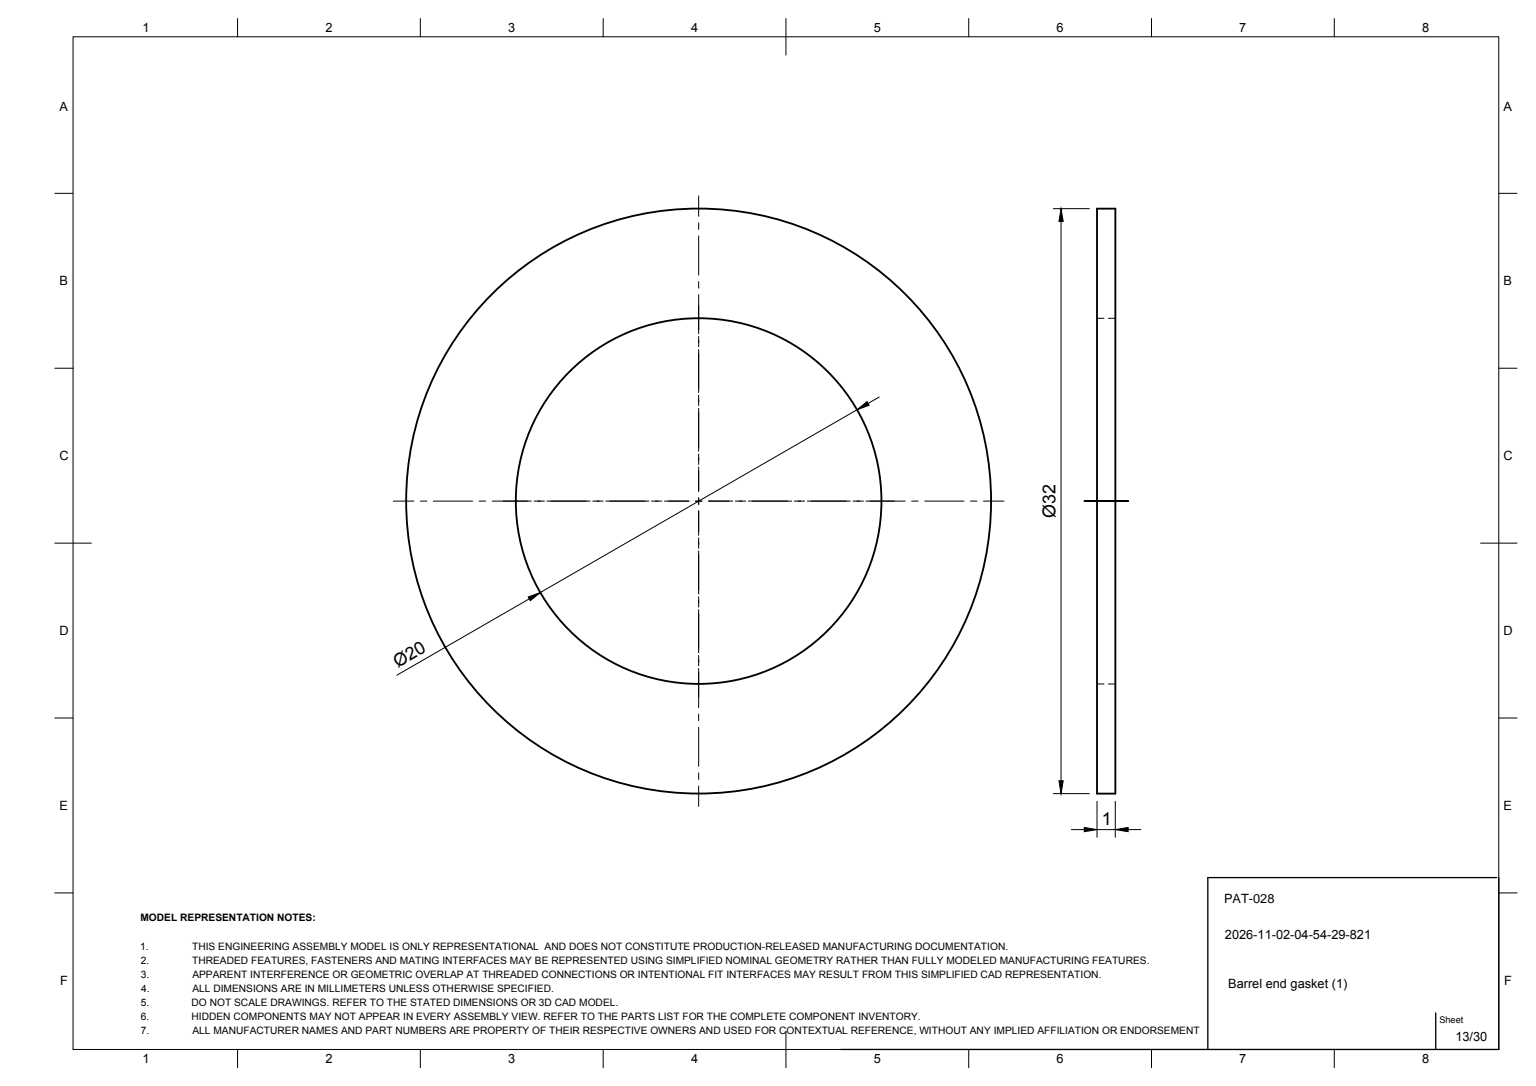
ISO-10303-21;
HEADER;
/* Generated by software containing ST-Developer
 * from STEP Tools, Inc. (www.steptools.com) 
 */

FILE_DESCRIPTION(
/* description */ ('Cylinder foot and clevis mount kit'),
/* implementation_level */ '2;1');

FILE_NAME(
/* name */ 'Barrel end gasket (1).step',
/* time_stamp */ '2026-10-27T20:10:43-07:00',
/* author */ (''),
/* organization */ (''),
/* preprocessor_version */ 'ST-DEVELOPER v20.2',
/* originating_system */ 'Autodesk Translation Framework v15.17.0.0',
/* authorisation */ '');

FILE_SCHEMA (('AUTOMOTIVE_DESIGN { 1 0 10303 214 3 1 1 }'));
ENDSEC;

DATA;
#10=MECHANICAL_DESIGN_GEOMETRIC_PRESENTATION_REPRESENTATION('',(#346),#9102);
#290=SHAPE_REPRESENTATION_RELATIONSHIP('SRR','None',#9237,#318);
#318=ADVANCED_BREP_SHAPE_REPRESENTATION('',(#374),#9080);
#346=STYLED_ITEM('',(#9453),#374);
#374=MANIFOLD_SOLID_BREP('Body1',#4932);
#444=FACE_BOUND('',#1197,.T.);
#445=FACE_BOUND('',#1199,.T.);
#595=PLANE('',#5539);
#596=PLANE('',#5540);
#836=FACE_OUTER_BOUND('',#1194,.T.);
#837=FACE_OUTER_BOUND('',#1195,.T.);
#838=FACE_OUTER_BOUND('',#1196,.T.);
#839=FACE_OUTER_BOUND('',#1198,.T.);
#1194=EDGE_LOOP('',(#3885,#3886,#3887,#3888));
#1195=EDGE_LOOP('',(#3889,#3890,#3891,#3892));
#1196=EDGE_LOOP('',(#3893));
#1197=EDGE_LOOP('',(#3894));
#1198=EDGE_LOOP('',(#3895));
#1199=EDGE_LOOP('',(#3896));
#1577=LINE('',#8115,#1926);
#1578=LINE('',#8121,#1927);
#1926=VECTOR('',#6602,1.);
#1927=VECTOR('',#6609,1.6);
#2212=CIRCLE('',#5534,1.);
#2213=CIRCLE('',#5535,1.);
#2214=CIRCLE('',#5537,1.6);
#2215=CIRCLE('',#5538,1.6);
#2506=VERTEX_POINT('',#8112);
#2507=VERTEX_POINT('',#8114);
#2508=VERTEX_POINT('',#8118);
#2509=VERTEX_POINT('',#8120);
#2997=EDGE_CURVE('',#2506,#2506,#2212,.T.);
#2998=EDGE_CURVE('',#2506,#2507,#1577,.T.);
#2999=EDGE_CURVE('',#2507,#2507,#2213,.T.);
#3000=EDGE_CURVE('',#2508,#2508,#2214,.T.);
#3001=EDGE_CURVE('',#2508,#2509,#1578,.T.);
#3002=EDGE_CURVE('',#2509,#2509,#2215,.T.);
#3885=ORIENTED_EDGE('',*,*,#2997,.F.);
#3886=ORIENTED_EDGE('',*,*,#2998,.T.);
#3887=ORIENTED_EDGE('',*,*,#2999,.T.);
#3888=ORIENTED_EDGE('',*,*,#2998,.F.);
#3889=ORIENTED_EDGE('',*,*,#3000,.F.);
#3890=ORIENTED_EDGE('',*,*,#3001,.T.);
#3891=ORIENTED_EDGE('',*,*,#3002,.T.);
#3892=ORIENTED_EDGE('',*,*,#3001,.F.);
#3893=ORIENTED_EDGE('',*,*,#3000,.T.);
#3894=ORIENTED_EDGE('',*,*,#2997,.T.);
#3895=ORIENTED_EDGE('',*,*,#3002,.F.);
#3896=ORIENTED_EDGE('',*,*,#2999,.F.);
#4572=CYLINDRICAL_SURFACE('',#5533,1.);
#4573=CYLINDRICAL_SURFACE('',#5536,1.6);
#4759=ADVANCED_FACE('',(#836),#4572,.F.);
#4760=ADVANCED_FACE('',(#837),#4573,.T.);
#4761=ADVANCED_FACE('',(#838,#444),#595,.T.);
#4762=ADVANCED_FACE('',(#839,#445),#596,.F.);
#4932=CLOSED_SHELL('',(#4759,#4760,#4761,#4762));
#5532=AXIS2_PLACEMENT_3D('',#8110,#6596,#6597);
#5533=AXIS2_PLACEMENT_3D('',#8111,#6598,#6599);
#5534=AXIS2_PLACEMENT_3D('',#8113,#6600,#6601);
#5535=AXIS2_PLACEMENT_3D('',#8116,#6603,#6604);
#5536=AXIS2_PLACEMENT_3D('',#8117,#6605,#6606);
#5537=AXIS2_PLACEMENT_3D('',#8119,#6607,#6608);
#5538=AXIS2_PLACEMENT_3D('',#8122,#6610,#6611);
#5539=AXIS2_PLACEMENT_3D('',#8123,#6612,#6613);
#5540=AXIS2_PLACEMENT_3D('',#8124,#6614,#6615);
#6596=DIRECTION('axis',(0.,0.,1.));
#6597=DIRECTION('refdir',(1.,0.,0.));
#6598=DIRECTION('center_axis',(0.,1.,0.));
#6599=DIRECTION('ref_axis',(1.,0.,0.));
#6600=DIRECTION('center_axis',(0.,-1.,0.));
#6601=DIRECTION('ref_axis',(1.,0.,0.));
#6602=DIRECTION('',(0.,-1.,0.));
#6603=DIRECTION('center_axis',(0.,-1.,0.));
#6604=DIRECTION('ref_axis',(1.,0.,0.));
#6605=DIRECTION('center_axis',(0.,1.,0.));
#6606=DIRECTION('ref_axis',(1.,0.,0.));
#6607=DIRECTION('center_axis',(0.,1.,0.));
#6608=DIRECTION('ref_axis',(1.,0.,0.));
#6609=DIRECTION('',(0.,-1.,0.));
#6610=DIRECTION('center_axis',(0.,1.,0.));
#6611=DIRECTION('ref_axis',(1.,0.,0.));
#6612=DIRECTION('center_axis',(0.,1.,0.));
#6613=DIRECTION('ref_axis',(1.,0.,0.));
#6614=DIRECTION('center_axis',(0.,1.,0.));
#6615=DIRECTION('ref_axis',(1.,0.,0.));
#8110=CARTESIAN_POINT('',(0.,0.,0.));
#8111=CARTESIAN_POINT('Origin',(0.,10.8,4.5));
#8112=CARTESIAN_POINT('',(-1.,10.9,4.5));
#8113=CARTESIAN_POINT('Origin',(0.,10.9,4.5));
#8114=CARTESIAN_POINT('',(-1.,10.8,4.5));
#8115=CARTESIAN_POINT('',(-1.,10.8,4.5));
#8116=CARTESIAN_POINT('Origin',(0.,10.8,4.5));
#8117=CARTESIAN_POINT('Origin',(0.,10.8,4.5));
#8118=CARTESIAN_POINT('',(-1.6,10.9,4.5));
#8119=CARTESIAN_POINT('Origin',(0.,10.9,4.5));
#8120=CARTESIAN_POINT('',(-1.6,10.8,4.5));
#8121=CARTESIAN_POINT('',(-1.6,10.8,4.5));
#8122=CARTESIAN_POINT('Origin',(0.,10.8,4.5));
#8123=CARTESIAN_POINT('Origin',(0.,10.9,4.5));
#8124=CARTESIAN_POINT('Origin',(0.,10.8,4.5));
#9047=UNCERTAINTY_MEASURE_WITH_UNIT(LENGTH_MEASURE(0.001),#9103,
'DISTANCE_ACCURACY_VALUE',
'Maximum model space distance between geometric entities at asserted c
onnectivities');
#9069=UNCERTAINTY_MEASURE_WITH_UNIT(LENGTH_MEASURE(0.001),#9103,
'DISTANCE_ACCURACY_VALUE',
'Maximum model space distance between geometric entities at asserted c
onnectivities');
#9080=(
GEOMETRIC_REPRESENTATION_CONTEXT(3)
GLOBAL_UNCERTAINTY_ASSIGNED_CONTEXT((#9047))
GLOBAL_UNIT_ASSIGNED_CONTEXT((#9103,#9105,#9106))
REPRESENTATION_CONTEXT('','3D')
);
#9102=(
GEOMETRIC_REPRESENTATION_CONTEXT(3)
GLOBAL_UNCERTAINTY_ASSIGNED_CONTEXT((#9069))
GLOBAL_UNIT_ASSIGNED_CONTEXT((#9103,#9105,#9106))
REPRESENTATION_CONTEXT('','3D')
);
#9103=(
LENGTH_UNIT()
NAMED_UNIT(*)
SI_UNIT(.CENTI.,.METRE.)
);
#9105=(
NAMED_UNIT(*)
PLANE_ANGLE_UNIT()
SI_UNIT($,.RADIAN.)
);
#9106=(
NAMED_UNIT(*)
SI_UNIT($,.STERADIAN.)
SOLID_ANGLE_UNIT()
);
#9117=SHAPE_DEFINITION_REPRESENTATION(#9149,#9237);
#9149=PRODUCT_DEFINITION_SHAPE('',$,#9270);
#9237=SHAPE_REPRESENTATION('',(#5532),#9080);
#9259=PRODUCT_DEFINITION_CONTEXT('part definition',#9357,'design');
#9270=PRODUCT_DEFINITION('Barrel end gasket (1)','Barrel end gasket (1)',
#9302,#9259);
#9302=PRODUCT_DEFINITION_FORMATION('',$,#9369);
#9357=APPLICATION_CONTEXT(
'Core Data for Automotive Mechanical Design Process');
#9358=PRODUCT_CONTEXT('part definition',#9357,'mechanical');
#9369=PRODUCT('Barrel end gasket (1)','Barrel end gasket (1)',
'Barrel end gasket (1)',(#9358));
#9447=COLOUR_RGB('Sky Blue',0.24,0.69,0.87);
#9448=FILL_AREA_STYLE_COLOUR('',#9447);
#9449=FILL_AREA_STYLE('',(#9448));
#9450=SURFACE_STYLE_FILL_AREA(#9449);
#9451=SURFACE_SIDE_STYLE('',(#9450));
#9452=SURFACE_STYLE_USAGE(.BOTH.,#9451);
#9453=PRESENTATION_STYLE_ASSIGNMENT((#9452));
ENDSEC;
END-ISO-10303-21;
